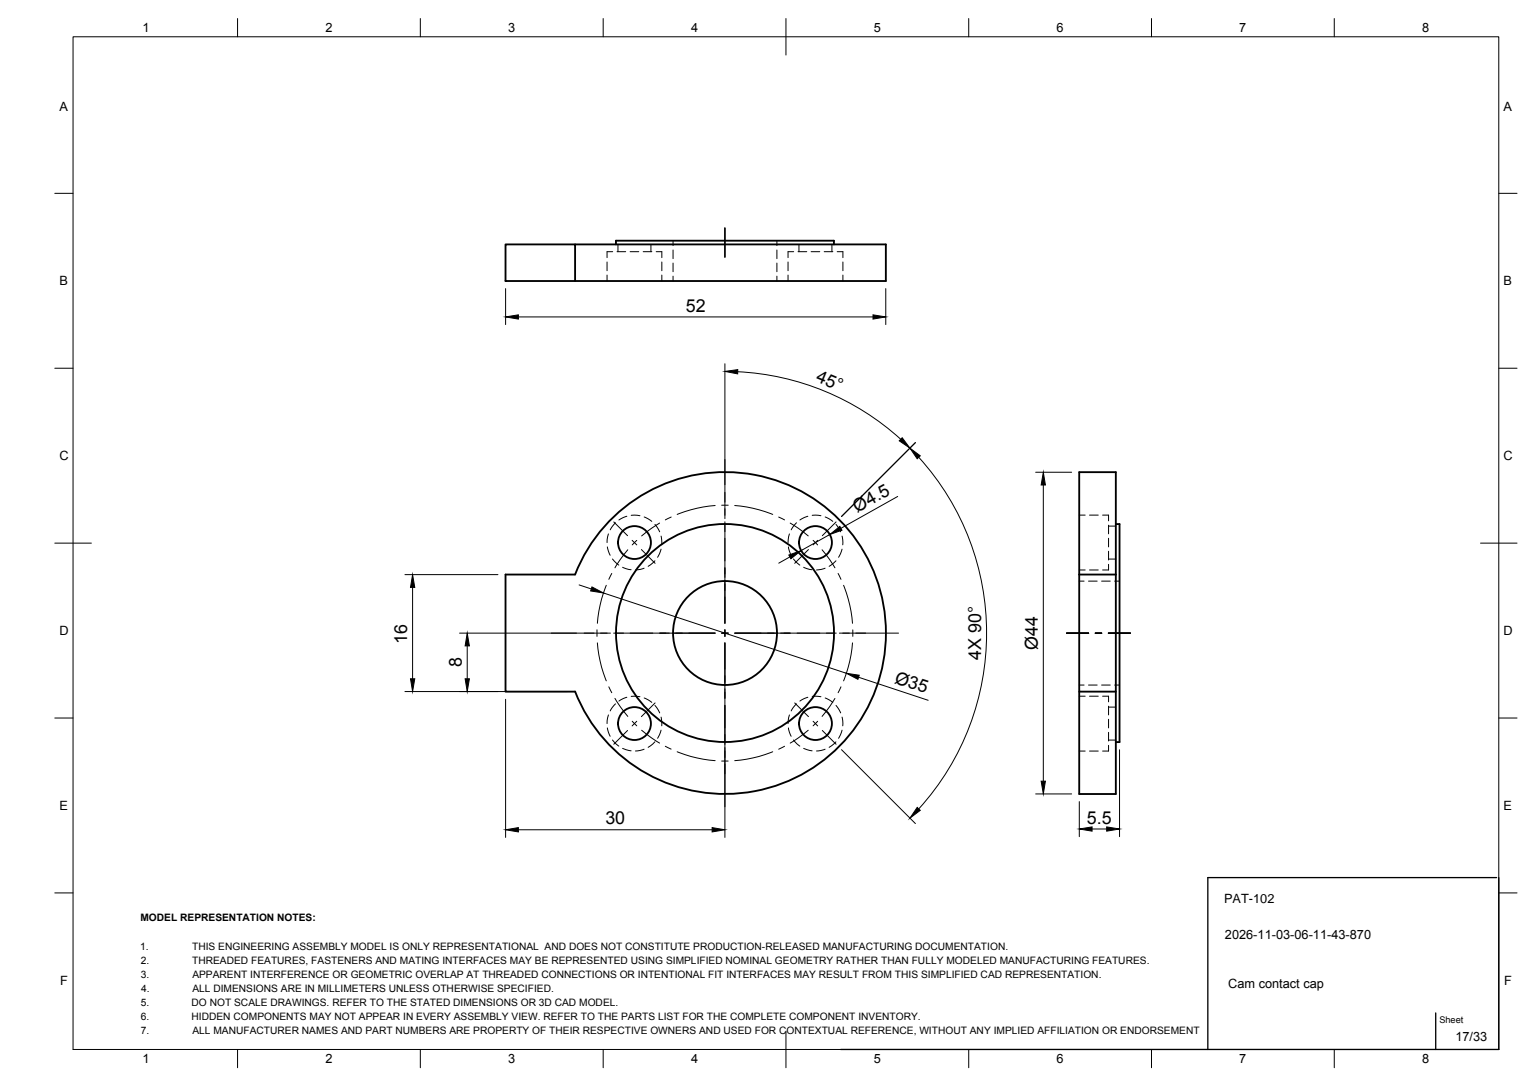
ISO-10303-21;
HEADER;
/* Generated by software containing ST-Developer
 * from STEP Tools, Inc. (www.steptools.com) 
 */

FILE_DESCRIPTION(
/* description */ ('Swing-away clamp arm'),
/* implementation_level */ '2;1');

FILE_NAME(
/* name */ 'Cam contact cap.step',
/* time_stamp */ '2026-10-28T03:26:03-07:00',
/* author */ (''),
/* organization */ (''),
/* preprocessor_version */ 'ST-DEVELOPER v20.2',
/* originating_system */ 'Autodesk Translation Framework v15.17.0.0',
/* authorisation */ '');

FILE_SCHEMA (('AUTOMOTIVE_DESIGN { 1 0 10303 214 3 1 1 }'));
ENDSEC;

DATA;
#10=MECHANICAL_DESIGN_GEOMETRIC_PRESENTATION_REPRESENTATION('',(#304),#10627);
#252=SHAPE_REPRESENTATION_RELATIONSHIP('SRR','None',#10751,#278);
#278=ADVANCED_BREP_SHAPE_REPRESENTATION('',(#337),#10610);
#304=STYLED_ITEM('',(#10951),#337);
#337=MANIFOLD_SOLID_BREP('Body1',#4911);
#416=FACE_BOUND('',#1161,.T.);
#417=FACE_BOUND('',#1164,.T.);
#418=FACE_BOUND('',#1167,.T.);
#419=FACE_BOUND('',#1170,.T.);
#420=FACE_BOUND('',#1180,.T.);
#421=FACE_BOUND('',#1184,.T.);
#422=FACE_BOUND('',#1185,.T.);
#423=FACE_BOUND('',#1186,.T.);
#424=FACE_BOUND('',#1187,.T.);
#425=FACE_BOUND('',#1188,.T.);
#426=FACE_BOUND('',#1190,.T.);
#427=FACE_BOUND('',#1191,.T.);
#428=FACE_BOUND('',#1192,.T.);
#429=FACE_BOUND('',#1193,.T.);
#430=FACE_BOUND('',#1194,.T.);
#563=PLANE('',#5523);
#564=PLANE('',#5528);
#565=PLANE('',#5533);
#566=PLANE('',#5538);
#567=PLANE('',#5548);
#568=PLANE('',#5549);
#569=PLANE('',#5550);
#570=PLANE('',#5554);
#571=PLANE('',#5561);
#572=PLANE('',#5562);
#794=FACE_OUTER_BOUND('',#1159,.T.);
#795=FACE_OUTER_BOUND('',#1160,.T.);
#796=FACE_OUTER_BOUND('',#1162,.T.);
#797=FACE_OUTER_BOUND('',#1163,.T.);
#798=FACE_OUTER_BOUND('',#1165,.T.);
#799=FACE_OUTER_BOUND('',#1166,.T.);
#800=FACE_OUTER_BOUND('',#1168,.T.);
#801=FACE_OUTER_BOUND('',#1169,.T.);
#802=FACE_OUTER_BOUND('',#1171,.T.);
#803=FACE_OUTER_BOUND('',#1172,.T.);
#804=FACE_OUTER_BOUND('',#1173,.T.);
#805=FACE_OUTER_BOUND('',#1174,.T.);
#806=FACE_OUTER_BOUND('',#1175,.T.);
#807=FACE_OUTER_BOUND('',#1176,.T.);
#808=FACE_OUTER_BOUND('',#1177,.T.);
#809=FACE_OUTER_BOUND('',#1178,.T.);
#810=FACE_OUTER_BOUND('',#1179,.T.);
#811=FACE_OUTER_BOUND('',#1181,.T.);
#812=FACE_OUTER_BOUND('',#1182,.T.);
#813=FACE_OUTER_BOUND('',#1183,.T.);
#814=FACE_OUTER_BOUND('',#1189,.T.);
#1159=EDGE_LOOP('',(#3939,#3940,#3941,#3942));
#1160=EDGE_LOOP('',(#3943));
#1161=EDGE_LOOP('',(#3944));
#1162=EDGE_LOOP('',(#3945,#3946,#3947,#3948));
#1163=EDGE_LOOP('',(#3949));
#1164=EDGE_LOOP('',(#3950));
#1165=EDGE_LOOP('',(#3951,#3952,#3953,#3954));
#1166=EDGE_LOOP('',(#3955));
#1167=EDGE_LOOP('',(#3956));
#1168=EDGE_LOOP('',(#3957,#3958,#3959,#3960));
#1169=EDGE_LOOP('',(#3961));
#1170=EDGE_LOOP('',(#3962));
#1171=EDGE_LOOP('',(#3963,#3964,#3965,#3966));
#1172=EDGE_LOOP('',(#3967,#3968,#3969,#3970));
#1173=EDGE_LOOP('',(#3971,#3972,#3973,#3974));
#1174=EDGE_LOOP('',(#3975,#3976,#3977,#3978));
#1175=EDGE_LOOP('',(#3979,#3980,#3981,#3982));
#1176=EDGE_LOOP('',(#3983,#3984,#3985,#3986));
#1177=EDGE_LOOP('',(#3987,#3988,#3989,#3990));
#1178=EDGE_LOOP('',(#3991,#3992,#3993,#3994));
#1179=EDGE_LOOP('',(#3995));
#1180=EDGE_LOOP('',(#3996));
#1181=EDGE_LOOP('',(#3997,#3998,#3999,#4000));
#1182=EDGE_LOOP('',(#4001,#4002,#4003,#4004));
#1183=EDGE_LOOP('',(#4005,#4006,#4007,#4008));
#1184=EDGE_LOOP('',(#4009));
#1185=EDGE_LOOP('',(#4010));
#1186=EDGE_LOOP('',(#4011));
#1187=EDGE_LOOP('',(#4012));
#1188=EDGE_LOOP('',(#4013));
#1189=EDGE_LOOP('',(#4014,#4015,#4016,#4017));
#1190=EDGE_LOOP('',(#4018));
#1191=EDGE_LOOP('',(#4019));
#1192=EDGE_LOOP('',(#4020));
#1193=EDGE_LOOP('',(#4021));
#1194=EDGE_LOOP('',(#4022));
#1563=LINE('',#9559,#1885);
#1564=LINE('',#9568,#1886);
#1565=LINE('',#9577,#1887);
#1566=LINE('',#9586,#1888);
#1567=LINE('',#9594,#1889);
#1568=LINE('',#9598,#1890);
#1569=LINE('',#9602,#1891);
#1570=LINE('',#9606,#1892);
#1571=LINE('',#9610,#1893);
#1572=LINE('',#9612,#1894);
#1573=LINE('',#9614,#1895);
#1574=LINE('',#9615,#1896);
#1575=LINE('',#9619,#1897);
#1576=LINE('',#9621,#1898);
#1577=LINE('',#9623,#1899);
#1578=LINE('',#9624,#1900);
#1579=LINE('',#9626,#1901);
#1580=LINE('',#9627,#1902);
#1581=LINE('',#9632,#1903);
#1582=LINE('',#9640,#1904);
#1885=VECTOR('',#6680,0.375);
#1886=VECTOR('',#6691,0.375);
#1887=VECTOR('',#6702,0.375);
#1888=VECTOR('',#6713,0.375);
#1889=VECTOR('',#6724,0.225);
#1890=VECTOR('',#6729,0.225);
#1891=VECTOR('',#6734,0.225);
#1892=VECTOR('',#6739,0.225);
#1893=VECTOR('',#6742,1.);
#1894=VECTOR('',#6743,1.);
#1895=VECTOR('',#6744,1.);
#1896=VECTOR('',#6745,1.);
#1897=VECTOR('',#6748,1.);
#1898=VECTOR('',#6749,1.);
#1899=VECTOR('',#6750,1.);
#1900=VECTOR('',#6751,1.);
#1901=VECTOR('',#6754,1.);
#1902=VECTOR('',#6755,1.);
#1903=VECTOR('',#6760,1.49);
#1904=VECTOR('',#6771,0.71);
#2111=CIRCLE('',#5521,0.375);
#2112=CIRCLE('',#5522,0.375);
#2113=CIRCLE('',#5524,0.225);
#2114=CIRCLE('',#5526,0.375);
#2115=CIRCLE('',#5527,0.375);
#2116=CIRCLE('',#5529,0.225);
#2117=CIRCLE('',#5531,0.375);
#2118=CIRCLE('',#5532,0.375);
#2119=CIRCLE('',#5534,0.225);
#2120=CIRCLE('',#5536,0.375);
#2121=CIRCLE('',#5537,0.375);
#2122=CIRCLE('',#5539,0.225);
#2123=CIRCLE('',#5541,0.225);
#2124=CIRCLE('',#5543,0.225);
#2125=CIRCLE('',#5545,0.225);
#2126=CIRCLE('',#5547,0.225);
#2127=CIRCLE('',#5552,1.49);
#2128=CIRCLE('',#5553,1.49);
#2129=CIRCLE('',#5555,0.71);
#2130=CIRCLE('',#5557,0.71);
#2131=CIRCLE('',#5559,2.2);
#2132=CIRCLE('',#5560,2.2);
#2480=VERTEX_POINT('',#9556);
#2481=VERTEX_POINT('',#9558);
#2482=VERTEX_POINT('',#9562);
#2483=VERTEX_POINT('',#9565);
#2484=VERTEX_POINT('',#9567);
#2485=VERTEX_POINT('',#9571);
#2486=VERTEX_POINT('',#9574);
#2487=VERTEX_POINT('',#9576);
#2488=VERTEX_POINT('',#9580);
#2489=VERTEX_POINT('',#9583);
#2490=VERTEX_POINT('',#9585);
#2491=VERTEX_POINT('',#9589);
#2492=VERTEX_POINT('',#9592);
#2493=VERTEX_POINT('',#9596);
#2494=VERTEX_POINT('',#9600);
#2495=VERTEX_POINT('',#9604);
#2496=VERTEX_POINT('',#9608);
#2497=VERTEX_POINT('',#9609);
#2498=VERTEX_POINT('',#9611);
#2499=VERTEX_POINT('',#9613);
#2500=VERTEX_POINT('',#9617);
#2501=VERTEX_POINT('',#9618);
#2502=VERTEX_POINT('',#9620);
#2503=VERTEX_POINT('',#9622);
#2504=VERTEX_POINT('',#9629);
#2505=VERTEX_POINT('',#9631);
#2506=VERTEX_POINT('',#9635);
#2507=VERTEX_POINT('',#9638);
#3002=EDGE_CURVE('',#2480,#2480,#2111,.T.);
#3003=EDGE_CURVE('',#2480,#2481,#1563,.T.);
#3004=EDGE_CURVE('',#2481,#2481,#2112,.T.);
#3005=EDGE_CURVE('',#2482,#2482,#2113,.T.);
#3006=EDGE_CURVE('',#2483,#2483,#2114,.T.);
#3007=EDGE_CURVE('',#2483,#2484,#1564,.T.);
#3008=EDGE_CURVE('',#2484,#2484,#2115,.T.);
#3009=EDGE_CURVE('',#2485,#2485,#2116,.T.);
#3010=EDGE_CURVE('',#2486,#2486,#2117,.T.);
#3011=EDGE_CURVE('',#2486,#2487,#1565,.T.);
#3012=EDGE_CURVE('',#2487,#2487,#2118,.T.);
#3013=EDGE_CURVE('',#2488,#2488,#2119,.T.);
#3014=EDGE_CURVE('',#2489,#2489,#2120,.T.);
#3015=EDGE_CURVE('',#2489,#2490,#1566,.T.);
#3016=EDGE_CURVE('',#2490,#2490,#2121,.T.);
#3017=EDGE_CURVE('',#2491,#2491,#2122,.T.);
#3018=EDGE_CURVE('',#2492,#2492,#2123,.T.);
#3019=EDGE_CURVE('',#2492,#2482,#1567,.T.);
#3020=EDGE_CURVE('',#2493,#2493,#2124,.T.);
#3021=EDGE_CURVE('',#2493,#2485,#1568,.T.);
#3022=EDGE_CURVE('',#2494,#2494,#2125,.T.);
#3023=EDGE_CURVE('',#2494,#2488,#1569,.T.);
#3024=EDGE_CURVE('',#2495,#2495,#2126,.T.);
#3025=EDGE_CURVE('',#2495,#2491,#1570,.T.);
#3026=EDGE_CURVE('',#2496,#2497,#1571,.T.);
#3027=EDGE_CURVE('',#2498,#2496,#1572,.T.);
#3028=EDGE_CURVE('',#2499,#2498,#1573,.T.);
#3029=EDGE_CURVE('',#2499,#2497,#1574,.T.);
#3030=EDGE_CURVE('',#2500,#2501,#1575,.T.);
#3031=EDGE_CURVE('',#2500,#2502,#1576,.T.);
#3032=EDGE_CURVE('',#2502,#2503,#1577,.T.);
#3033=EDGE_CURVE('',#2501,#2503,#1578,.T.);
#3034=EDGE_CURVE('',#2502,#2499,#1579,.T.);
#3035=EDGE_CURVE('',#2503,#2498,#1580,.T.);
#3036=EDGE_CURVE('',#2504,#2504,#2127,.T.);
#3037=EDGE_CURVE('',#2504,#2505,#1581,.T.);
#3038=EDGE_CURVE('',#2505,#2505,#2128,.T.);
#3039=EDGE_CURVE('',#2506,#2506,#2129,.T.);
#3040=EDGE_CURVE('',#2507,#2507,#2130,.T.);
#3041=EDGE_CURVE('',#2507,#2506,#1582,.T.);
#3042=EDGE_CURVE('',#2497,#2500,#2131,.T.);
#3043=EDGE_CURVE('',#2496,#2501,#2132,.T.);
#3939=ORIENTED_EDGE('',*,*,#3002,.F.);
#3940=ORIENTED_EDGE('',*,*,#3003,.T.);
#3941=ORIENTED_EDGE('',*,*,#3004,.F.);
#3942=ORIENTED_EDGE('',*,*,#3003,.F.);
#3943=ORIENTED_EDGE('',*,*,#3002,.T.);
#3944=ORIENTED_EDGE('',*,*,#3005,.F.);
#3945=ORIENTED_EDGE('',*,*,#3006,.F.);
#3946=ORIENTED_EDGE('',*,*,#3007,.T.);
#3947=ORIENTED_EDGE('',*,*,#3008,.F.);
#3948=ORIENTED_EDGE('',*,*,#3007,.F.);
#3949=ORIENTED_EDGE('',*,*,#3006,.T.);
#3950=ORIENTED_EDGE('',*,*,#3009,.F.);
#3951=ORIENTED_EDGE('',*,*,#3010,.F.);
#3952=ORIENTED_EDGE('',*,*,#3011,.T.);
#3953=ORIENTED_EDGE('',*,*,#3012,.F.);
#3954=ORIENTED_EDGE('',*,*,#3011,.F.);
#3955=ORIENTED_EDGE('',*,*,#3010,.T.);
#3956=ORIENTED_EDGE('',*,*,#3013,.F.);
#3957=ORIENTED_EDGE('',*,*,#3014,.F.);
#3958=ORIENTED_EDGE('',*,*,#3015,.T.);
#3959=ORIENTED_EDGE('',*,*,#3016,.F.);
#3960=ORIENTED_EDGE('',*,*,#3015,.F.);
#3961=ORIENTED_EDGE('',*,*,#3014,.T.);
#3962=ORIENTED_EDGE('',*,*,#3017,.F.);
#3963=ORIENTED_EDGE('',*,*,#3018,.F.);
#3964=ORIENTED_EDGE('',*,*,#3019,.T.);
#3965=ORIENTED_EDGE('',*,*,#3005,.T.);
#3966=ORIENTED_EDGE('',*,*,#3019,.F.);
#3967=ORIENTED_EDGE('',*,*,#3020,.F.);
#3968=ORIENTED_EDGE('',*,*,#3021,.T.);
#3969=ORIENTED_EDGE('',*,*,#3009,.T.);
#3970=ORIENTED_EDGE('',*,*,#3021,.F.);
#3971=ORIENTED_EDGE('',*,*,#3022,.F.);
#3972=ORIENTED_EDGE('',*,*,#3023,.T.);
#3973=ORIENTED_EDGE('',*,*,#3013,.T.);
#3974=ORIENTED_EDGE('',*,*,#3023,.F.);
#3975=ORIENTED_EDGE('',*,*,#3024,.F.);
#3976=ORIENTED_EDGE('',*,*,#3025,.T.);
#3977=ORIENTED_EDGE('',*,*,#3017,.T.);
#3978=ORIENTED_EDGE('',*,*,#3025,.F.);
#3979=ORIENTED_EDGE('',*,*,#3026,.F.);
#3980=ORIENTED_EDGE('',*,*,#3027,.F.);
#3981=ORIENTED_EDGE('',*,*,#3028,.F.);
#3982=ORIENTED_EDGE('',*,*,#3029,.T.);
#3983=ORIENTED_EDGE('',*,*,#3030,.F.);
#3984=ORIENTED_EDGE('',*,*,#3031,.T.);
#3985=ORIENTED_EDGE('',*,*,#3032,.T.);
#3986=ORIENTED_EDGE('',*,*,#3033,.F.);
#3987=ORIENTED_EDGE('',*,*,#3034,.T.);
#3988=ORIENTED_EDGE('',*,*,#3028,.T.);
#3989=ORIENTED_EDGE('',*,*,#3035,.F.);
#3990=ORIENTED_EDGE('',*,*,#3032,.F.);
#3991=ORIENTED_EDGE('',*,*,#3036,.F.);
#3992=ORIENTED_EDGE('',*,*,#3037,.T.);
#3993=ORIENTED_EDGE('',*,*,#3038,.T.);
#3994=ORIENTED_EDGE('',*,*,#3037,.F.);
#3995=ORIENTED_EDGE('',*,*,#3038,.F.);
#3996=ORIENTED_EDGE('',*,*,#3039,.F.);
#3997=ORIENTED_EDGE('',*,*,#3040,.F.);
#3998=ORIENTED_EDGE('',*,*,#3041,.T.);
#3999=ORIENTED_EDGE('',*,*,#3039,.T.);
#4000=ORIENTED_EDGE('',*,*,#3041,.F.);
#4001=ORIENTED_EDGE('',*,*,#3026,.T.);
#4002=ORIENTED_EDGE('',*,*,#3042,.T.);
#4003=ORIENTED_EDGE('',*,*,#3030,.T.);
#4004=ORIENTED_EDGE('',*,*,#3043,.F.);
#4005=ORIENTED_EDGE('',*,*,#3043,.T.);
#4006=ORIENTED_EDGE('',*,*,#3033,.T.);
#4007=ORIENTED_EDGE('',*,*,#3035,.T.);
#4008=ORIENTED_EDGE('',*,*,#3027,.T.);
#4009=ORIENTED_EDGE('',*,*,#3040,.T.);
#4010=ORIENTED_EDGE('',*,*,#3016,.T.);
#4011=ORIENTED_EDGE('',*,*,#3012,.T.);
#4012=ORIENTED_EDGE('',*,*,#3008,.T.);
#4013=ORIENTED_EDGE('',*,*,#3004,.T.);
#4014=ORIENTED_EDGE('',*,*,#3042,.F.);
#4015=ORIENTED_EDGE('',*,*,#3029,.F.);
#4016=ORIENTED_EDGE('',*,*,#3034,.F.);
#4017=ORIENTED_EDGE('',*,*,#3031,.F.);
#4018=ORIENTED_EDGE('',*,*,#3036,.T.);
#4019=ORIENTED_EDGE('',*,*,#3024,.T.);
#4020=ORIENTED_EDGE('',*,*,#3022,.T.);
#4021=ORIENTED_EDGE('',*,*,#3020,.T.);
#4022=ORIENTED_EDGE('',*,*,#3018,.T.);
#4545=CYLINDRICAL_SURFACE('',#5520,0.375);
#4546=CYLINDRICAL_SURFACE('',#5525,0.375);
#4547=CYLINDRICAL_SURFACE('',#5530,0.375);
#4548=CYLINDRICAL_SURFACE('',#5535,0.375);
#4549=CYLINDRICAL_SURFACE('',#5540,0.225);
#4550=CYLINDRICAL_SURFACE('',#5542,0.225);
#4551=CYLINDRICAL_SURFACE('',#5544,0.225);
#4552=CYLINDRICAL_SURFACE('',#5546,0.225);
#4553=CYLINDRICAL_SURFACE('',#5551,1.49);
#4554=CYLINDRICAL_SURFACE('',#5556,0.71);
#4555=CYLINDRICAL_SURFACE('',#5558,2.2);
#4749=ADVANCED_FACE('',(#794),#4545,.F.);
#4750=ADVANCED_FACE('',(#795,#416),#563,.T.);
#4751=ADVANCED_FACE('',(#796),#4546,.F.);
#4752=ADVANCED_FACE('',(#797,#417),#564,.T.);
#4753=ADVANCED_FACE('',(#798),#4547,.F.);
#4754=ADVANCED_FACE('',(#799,#418),#565,.T.);
#4755=ADVANCED_FACE('',(#800),#4548,.F.);
#4756=ADVANCED_FACE('',(#801,#419),#566,.T.);
#4757=ADVANCED_FACE('',(#802),#4549,.F.);
#4758=ADVANCED_FACE('',(#803),#4550,.F.);
#4759=ADVANCED_FACE('',(#804),#4551,.F.);
#4760=ADVANCED_FACE('',(#805),#4552,.F.);
#4761=ADVANCED_FACE('',(#806),#567,.T.);
#4762=ADVANCED_FACE('',(#807),#568,.T.);
#4763=ADVANCED_FACE('',(#808),#569,.T.);
#4764=ADVANCED_FACE('',(#809),#4553,.T.);
#4765=ADVANCED_FACE('',(#810,#420),#570,.F.);
#4766=ADVANCED_FACE('',(#811),#4554,.F.);
#4767=ADVANCED_FACE('',(#812),#4555,.T.);
#4768=ADVANCED_FACE('',(#813,#421,#422,#423,#424,#425),#571,.T.);
#4769=ADVANCED_FACE('',(#814,#426,#427,#428,#429,#430),#572,.F.);
#4911=CLOSED_SHELL('',(#4749,#4750,#4751,#4752,#4753,#4754,#4755,#4756,
#4757,#4758,#4759,#4760,#4761,#4762,#4763,#4764,#4765,#4766,#4767,#4768,
#4769));
#5519=AXIS2_PLACEMENT_3D('',#9554,#6674,#6675);
#5520=AXIS2_PLACEMENT_3D('',#9555,#6676,#6677);
#5521=AXIS2_PLACEMENT_3D('',#9557,#6678,#6679);
#5522=AXIS2_PLACEMENT_3D('',#9560,#6681,#6682);
#5523=AXIS2_PLACEMENT_3D('',#9561,#6683,#6684);
#5524=AXIS2_PLACEMENT_3D('',#9563,#6685,#6686);
#5525=AXIS2_PLACEMENT_3D('',#9564,#6687,#6688);
#5526=AXIS2_PLACEMENT_3D('',#9566,#6689,#6690);
#5527=AXIS2_PLACEMENT_3D('',#9569,#6692,#6693);
#5528=AXIS2_PLACEMENT_3D('',#9570,#6694,#6695);
#5529=AXIS2_PLACEMENT_3D('',#9572,#6696,#6697);
#5530=AXIS2_PLACEMENT_3D('',#9573,#6698,#6699);
#5531=AXIS2_PLACEMENT_3D('',#9575,#6700,#6701);
#5532=AXIS2_PLACEMENT_3D('',#9578,#6703,#6704);
#5533=AXIS2_PLACEMENT_3D('',#9579,#6705,#6706);
#5534=AXIS2_PLACEMENT_3D('',#9581,#6707,#6708);
#5535=AXIS2_PLACEMENT_3D('',#9582,#6709,#6710);
#5536=AXIS2_PLACEMENT_3D('',#9584,#6711,#6712);
#5537=AXIS2_PLACEMENT_3D('',#9587,#6714,#6715);
#5538=AXIS2_PLACEMENT_3D('',#9588,#6716,#6717);
#5539=AXIS2_PLACEMENT_3D('',#9590,#6718,#6719);
#5540=AXIS2_PLACEMENT_3D('',#9591,#6720,#6721);
#5541=AXIS2_PLACEMENT_3D('',#9593,#6722,#6723);
#5542=AXIS2_PLACEMENT_3D('',#9595,#6725,#6726);
#5543=AXIS2_PLACEMENT_3D('',#9597,#6727,#6728);
#5544=AXIS2_PLACEMENT_3D('',#9599,#6730,#6731);
#5545=AXIS2_PLACEMENT_3D('',#9601,#6732,#6733);
#5546=AXIS2_PLACEMENT_3D('',#9603,#6735,#6736);
#5547=AXIS2_PLACEMENT_3D('',#9605,#6737,#6738);
#5548=AXIS2_PLACEMENT_3D('',#9607,#6740,#6741);
#5549=AXIS2_PLACEMENT_3D('',#9616,#6746,#6747);
#5550=AXIS2_PLACEMENT_3D('',#9625,#6752,#6753);
#5551=AXIS2_PLACEMENT_3D('',#9628,#6756,#6757);
#5552=AXIS2_PLACEMENT_3D('',#9630,#6758,#6759);
#5553=AXIS2_PLACEMENT_3D('',#9633,#6761,#6762);
#5554=AXIS2_PLACEMENT_3D('',#9634,#6763,#6764);
#5555=AXIS2_PLACEMENT_3D('',#9636,#6765,#6766);
#5556=AXIS2_PLACEMENT_3D('',#9637,#6767,#6768);
#5557=AXIS2_PLACEMENT_3D('',#9639,#6769,#6770);
#5558=AXIS2_PLACEMENT_3D('',#9641,#6772,#6773);
#5559=AXIS2_PLACEMENT_3D('',#9642,#6774,#6775);
#5560=AXIS2_PLACEMENT_3D('',#9643,#6776,#6777);
#5561=AXIS2_PLACEMENT_3D('',#9644,#6778,#6779);
#5562=AXIS2_PLACEMENT_3D('',#9645,#6780,#6781);
#6674=DIRECTION('axis',(0.,0.,1.));
#6675=DIRECTION('refdir',(1.,0.,0.));
#6676=DIRECTION('center_axis',(0.,0.,1.));
#6677=DIRECTION('ref_axis',(1.,0.,0.));
#6678=DIRECTION('center_axis',(0.,0.,1.));
#6679=DIRECTION('ref_axis',(1.,0.,0.));
#6680=DIRECTION('',(0.,0.,1.));
#6681=DIRECTION('center_axis',(0.,0.,-1.));
#6682=DIRECTION('ref_axis',(1.,0.,0.));
#6683=DIRECTION('center_axis',(0.,0.,1.));
#6684=DIRECTION('ref_axis',(1.,0.,0.));
#6685=DIRECTION('center_axis',(0.,0.,1.));
#6686=DIRECTION('ref_axis',(1.,0.,0.));
#6687=DIRECTION('center_axis',(0.,0.,1.));
#6688=DIRECTION('ref_axis',(1.,0.,0.));
#6689=DIRECTION('center_axis',(0.,0.,1.));
#6690=DIRECTION('ref_axis',(1.,0.,0.));
#6691=DIRECTION('',(0.,0.,1.));
#6692=DIRECTION('center_axis',(0.,0.,-1.));
#6693=DIRECTION('ref_axis',(1.,0.,0.));
#6694=DIRECTION('center_axis',(0.,0.,1.));
#6695=DIRECTION('ref_axis',(1.,0.,0.));
#6696=DIRECTION('center_axis',(0.,0.,1.));
#6697=DIRECTION('ref_axis',(1.,0.,0.));
#6698=DIRECTION('center_axis',(0.,0.,1.));
#6699=DIRECTION('ref_axis',(1.,0.,0.));
#6700=DIRECTION('center_axis',(0.,0.,1.));
#6701=DIRECTION('ref_axis',(1.,0.,0.));
#6702=DIRECTION('',(0.,0.,1.));
#6703=DIRECTION('center_axis',(0.,0.,-1.));
#6704=DIRECTION('ref_axis',(1.,0.,0.));
#6705=DIRECTION('center_axis',(0.,0.,1.));
#6706=DIRECTION('ref_axis',(1.,0.,0.));
#6707=DIRECTION('center_axis',(0.,0.,1.));
#6708=DIRECTION('ref_axis',(1.,0.,0.));
#6709=DIRECTION('center_axis',(0.,0.,1.));
#6710=DIRECTION('ref_axis',(1.,0.,0.));
#6711=DIRECTION('center_axis',(0.,0.,1.));
#6712=DIRECTION('ref_axis',(1.,0.,0.));
#6713=DIRECTION('',(0.,0.,1.));
#6714=DIRECTION('center_axis',(0.,0.,-1.));
#6715=DIRECTION('ref_axis',(1.,0.,0.));
#6716=DIRECTION('center_axis',(0.,0.,1.));
#6717=DIRECTION('ref_axis',(1.,0.,0.));
#6718=DIRECTION('center_axis',(0.,0.,1.));
#6719=DIRECTION('ref_axis',(1.,0.,0.));
#6720=DIRECTION('center_axis',(0.,0.,1.));
#6721=DIRECTION('ref_axis',(1.,0.,0.));
#6722=DIRECTION('center_axis',(0.,0.,1.));
#6723=DIRECTION('ref_axis',(1.,0.,0.));
#6724=DIRECTION('',(0.,0.,1.));
#6725=DIRECTION('center_axis',(0.,0.,1.));
#6726=DIRECTION('ref_axis',(1.,0.,0.));
#6727=DIRECTION('center_axis',(0.,0.,1.));
#6728=DIRECTION('ref_axis',(1.,0.,0.));
#6729=DIRECTION('',(0.,0.,1.));
#6730=DIRECTION('center_axis',(0.,0.,1.));
#6731=DIRECTION('ref_axis',(1.,0.,0.));
#6732=DIRECTION('center_axis',(0.,0.,1.));
#6733=DIRECTION('ref_axis',(1.,0.,0.));
#6734=DIRECTION('',(0.,0.,1.));
#6735=DIRECTION('center_axis',(0.,0.,1.));
#6736=DIRECTION('ref_axis',(1.,0.,0.));
#6737=DIRECTION('center_axis',(0.,0.,1.));
#6738=DIRECTION('ref_axis',(1.,0.,0.));
#6739=DIRECTION('',(0.,0.,1.));
#6740=DIRECTION('center_axis',(0.,1.,0.));
#6741=DIRECTION('ref_axis',(-1.,0.,0.));
#6742=DIRECTION('',(0.,0.,-1.));
#6743=DIRECTION('',(-1.,0.,0.));
#6744=DIRECTION('',(0.,0.,1.));
#6745=DIRECTION('',(-1.,0.,0.));
#6746=DIRECTION('center_axis',(0.,-1.,0.));
#6747=DIRECTION('ref_axis',(1.,0.,0.));
#6748=DIRECTION('',(0.,0.,1.));
#6749=DIRECTION('',(1.,0.,0.));
#6750=DIRECTION('',(0.,0.,1.));
#6751=DIRECTION('',(1.,0.,0.));
#6752=DIRECTION('center_axis',(1.,0.,0.));
#6753=DIRECTION('ref_axis',(0.,1.,0.));
#6754=DIRECTION('',(0.,1.,0.));
#6755=DIRECTION('',(0.,1.,0.));
#6756=DIRECTION('center_axis',(0.,0.,1.));
#6757=DIRECTION('ref_axis',(1.,0.,0.));
#6758=DIRECTION('center_axis',(0.,0.,1.));
#6759=DIRECTION('ref_axis',(1.,0.,0.));
#6760=DIRECTION('',(0.,0.,-1.));
#6761=DIRECTION('center_axis',(0.,0.,1.));
#6762=DIRECTION('ref_axis',(1.,0.,0.));
#6763=DIRECTION('center_axis',(0.,0.,1.));
#6764=DIRECTION('ref_axis',(1.,0.,0.));
#6765=DIRECTION('center_axis',(0.,0.,-1.));
#6766=DIRECTION('ref_axis',(1.,0.,0.));
#6767=DIRECTION('center_axis',(0.,0.,1.));
#6768=DIRECTION('ref_axis',(1.,0.,0.));
#6769=DIRECTION('center_axis',(0.,0.,-1.));
#6770=DIRECTION('ref_axis',(1.,0.,0.));
#6771=DIRECTION('',(0.,0.,-1.));
#6772=DIRECTION('center_axis',(0.,0.,1.));
#6773=DIRECTION('ref_axis',(-1.,1.22464679914735E-16,0.));
#6774=DIRECTION('center_axis',(0.,0.,1.));
#6775=DIRECTION('ref_axis',(1.,0.,0.));
#6776=DIRECTION('center_axis',(0.,0.,1.));
#6777=DIRECTION('ref_axis',(1.,0.,0.));
#6778=DIRECTION('center_axis',(0.,0.,1.));
#6779=DIRECTION('ref_axis',(1.,0.,0.));
#6780=DIRECTION('center_axis',(0.,0.,1.));
#6781=DIRECTION('ref_axis',(1.,0.,0.));
#9554=CARTESIAN_POINT('',(0.,0.,0.));
#9555=CARTESIAN_POINT('Origin',(-1.23743686707646,-1.23743686707646,9.1));
#9556=CARTESIAN_POINT('',(-1.61243686707646,-1.23743686707646,9.1));
#9557=CARTESIAN_POINT('Origin',(-1.23743686707646,-1.23743686707646,9.1));
#9558=CARTESIAN_POINT('',(-1.61243686707646,-1.23743686707646,9.5));
#9559=CARTESIAN_POINT('',(-1.61243686707646,-1.23743686707646,9.1));
#9560=CARTESIAN_POINT('Origin',(-1.23743686707646,-1.23743686707646,9.5));
#9561=CARTESIAN_POINT('Origin',(-1.23743686707646,-1.23743686707646,9.1));
#9562=CARTESIAN_POINT('',(-1.46243686707646,-1.23743686707646,9.1));
#9563=CARTESIAN_POINT('Origin',(-1.23743686707646,-1.23743686707646,9.1));
#9564=CARTESIAN_POINT('Origin',(-1.23743686707646,1.23743686707646,9.1));
#9565=CARTESIAN_POINT('',(-1.61243686707646,1.23743686707646,9.1));
#9566=CARTESIAN_POINT('Origin',(-1.23743686707646,1.23743686707646,9.1));
#9567=CARTESIAN_POINT('',(-1.61243686707646,1.23743686707646,9.5));
#9568=CARTESIAN_POINT('',(-1.61243686707646,1.23743686707646,9.1));
#9569=CARTESIAN_POINT('Origin',(-1.23743686707646,1.23743686707646,9.5));
#9570=CARTESIAN_POINT('Origin',(-1.23743686707646,1.23743686707646,9.1));
#9571=CARTESIAN_POINT('',(-1.46243686707646,1.23743686707646,9.1));
#9572=CARTESIAN_POINT('Origin',(-1.23743686707646,1.23743686707646,9.1));
#9573=CARTESIAN_POINT('Origin',(1.23743686707646,1.23743686707646,9.1));
#9574=CARTESIAN_POINT('',(0.862436867076458,1.23743686707646,9.1));
#9575=CARTESIAN_POINT('Origin',(1.23743686707646,1.23743686707646,9.1));
#9576=CARTESIAN_POINT('',(0.862436867076458,1.23743686707646,9.5));
#9577=CARTESIAN_POINT('',(0.862436867076458,1.23743686707646,9.1));
#9578=CARTESIAN_POINT('Origin',(1.23743686707646,1.23743686707646,9.5));
#9579=CARTESIAN_POINT('Origin',(1.23743686707646,1.23743686707646,9.1));
#9580=CARTESIAN_POINT('',(1.01243686707646,1.23743686707646,9.1));
#9581=CARTESIAN_POINT('Origin',(1.23743686707646,1.23743686707646,9.1));
#9582=CARTESIAN_POINT('Origin',(1.23743686707646,-1.23743686707646,9.1));
#9583=CARTESIAN_POINT('',(0.862436867076458,-1.23743686707646,9.1));
#9584=CARTESIAN_POINT('Origin',(1.23743686707646,-1.23743686707646,9.1));
#9585=CARTESIAN_POINT('',(0.862436867076458,-1.23743686707646,9.5));
#9586=CARTESIAN_POINT('',(0.862436867076458,-1.23743686707646,9.1));
#9587=CARTESIAN_POINT('Origin',(1.23743686707646,-1.23743686707646,9.5));
#9588=CARTESIAN_POINT('Origin',(1.23743686707646,-1.23743686707646,9.1));
#9589=CARTESIAN_POINT('',(1.01243686707646,-1.23743686707646,9.1));
#9590=CARTESIAN_POINT('Origin',(1.23743686707646,-1.23743686707646,9.1));
#9591=CARTESIAN_POINT('Origin',(-1.23743686707646,-1.23743686707646,8.9));
#9592=CARTESIAN_POINT('',(-1.46243686707646,-1.23743686707646,9.));
#9593=CARTESIAN_POINT('Origin',(-1.23743686707646,-1.23743686707646,9.));
#9594=CARTESIAN_POINT('',(-1.46243686707646,-1.23743686707646,8.9));
#9595=CARTESIAN_POINT('Origin',(-1.23743686707646,1.23743686707646,8.9));
#9596=CARTESIAN_POINT('',(-1.46243686707646,1.23743686707646,9.));
#9597=CARTESIAN_POINT('Origin',(-1.23743686707646,1.23743686707646,9.));
#9598=CARTESIAN_POINT('',(-1.46243686707646,1.23743686707646,8.9));
#9599=CARTESIAN_POINT('Origin',(1.23743686707646,1.23743686707646,8.9));
#9600=CARTESIAN_POINT('',(1.01243686707646,1.23743686707646,9.));
#9601=CARTESIAN_POINT('Origin',(1.23743686707646,1.23743686707646,9.));
#9602=CARTESIAN_POINT('',(1.01243686707646,1.23743686707646,8.9));
#9603=CARTESIAN_POINT('Origin',(1.23743686707646,-1.23743686707646,8.9));
#9604=CARTESIAN_POINT('',(1.01243686707646,-1.23743686707646,9.));
#9605=CARTESIAN_POINT('Origin',(1.23743686707646,-1.23743686707646,9.));
#9606=CARTESIAN_POINT('',(1.01243686707646,-1.23743686707646,8.9));
#9607=CARTESIAN_POINT('Origin',(3.,0.8,9.));
#9608=CARTESIAN_POINT('',(2.04939015319192,0.8,9.5));
#9609=CARTESIAN_POINT('',(2.04939015319192,0.8,9.));
#9610=CARTESIAN_POINT('',(2.04939015319192,0.8,9.));
#9611=CARTESIAN_POINT('',(3.,0.8,9.5));
#9612=CARTESIAN_POINT('',(3.,0.8,9.5));
#9613=CARTESIAN_POINT('',(3.,0.8,9.));
#9614=CARTESIAN_POINT('',(3.,0.8,9.));
#9615=CARTESIAN_POINT('',(3.,0.8,9.));
#9616=CARTESIAN_POINT('Origin',(1.2,-0.8,9.));
#9617=CARTESIAN_POINT('',(2.04939015319192,-0.8,9.));
#9618=CARTESIAN_POINT('',(2.04939015319192,-0.8,9.5));
#9619=CARTESIAN_POINT('',(2.04939015319192,-0.8,9.));
#9620=CARTESIAN_POINT('',(3.,-0.8,9.));
#9621=CARTESIAN_POINT('',(1.2,-0.8,9.));
#9622=CARTESIAN_POINT('',(3.,-0.8,9.5));
#9623=CARTESIAN_POINT('',(3.,-0.8,9.));
#9624=CARTESIAN_POINT('',(1.2,-0.8,9.5));
#9625=CARTESIAN_POINT('Origin',(3.,-0.8,9.));
#9626=CARTESIAN_POINT('',(3.,-0.8,9.));
#9627=CARTESIAN_POINT('',(3.,-0.8,9.5));
#9628=CARTESIAN_POINT('Origin',(0.,0.,8.95));
#9629=CARTESIAN_POINT('',(-1.49,-1.82472373072956E-16,9.));
#9630=CARTESIAN_POINT('Origin',(0.,0.,9.));
#9631=CARTESIAN_POINT('',(-1.49,-1.82472373072956E-16,8.95));
#9632=CARTESIAN_POINT('',(-1.49,-1.82472373072956E-16,8.95));
#9633=CARTESIAN_POINT('Origin',(0.,0.,8.95));
#9634=CARTESIAN_POINT('Origin',(0.,0.,8.95));
#9635=CARTESIAN_POINT('',(-0.71,-8.69499227394621E-17,8.95));
#9636=CARTESIAN_POINT('Origin',(0.,0.,8.95));
#9637=CARTESIAN_POINT('Origin',(0.,0.,9.));
#9638=CARTESIAN_POINT('',(-0.71,-8.69499227394621E-17,9.5));
#9639=CARTESIAN_POINT('Origin',(0.,0.,9.5));
#9640=CARTESIAN_POINT('',(-0.71,-8.69499227394621E-17,9.));
#9641=CARTESIAN_POINT('Origin',(0.,0.,9.));
#9642=CARTESIAN_POINT('Origin',(0.,0.,9.));
#9643=CARTESIAN_POINT('Origin',(0.,0.,9.5));
#9644=CARTESIAN_POINT('Origin',(0.,0.,9.5));
#9645=CARTESIAN_POINT('Origin',(0.,0.,9.));
#10578=UNCERTAINTY_MEASURE_WITH_UNIT(LENGTH_MEASURE(0.001),#10628,
'DISTANCE_ACCURACY_VALUE',
'Maximum model space distance between geometric entities at asserted c
onnectivities');
#10595=UNCERTAINTY_MEASURE_WITH_UNIT(LENGTH_MEASURE(0.001),#10628,
'DISTANCE_ACCURACY_VALUE',
'Maximum model space distance between geometric entities at asserted c
onnectivities');
#10610=(
GEOMETRIC_REPRESENTATION_CONTEXT(3)
GLOBAL_UNCERTAINTY_ASSIGNED_CONTEXT((#10578))
GLOBAL_UNIT_ASSIGNED_CONTEXT((#10628,#10630,#10631))
REPRESENTATION_CONTEXT('','3D')
);
#10627=(
GEOMETRIC_REPRESENTATION_CONTEXT(3)
GLOBAL_UNCERTAINTY_ASSIGNED_CONTEXT((#10595))
GLOBAL_UNIT_ASSIGNED_CONTEXT((#10628,#10630,#10631))
REPRESENTATION_CONTEXT('','3D')
);
#10628=(
LENGTH_UNIT()
NAMED_UNIT(*)
SI_UNIT(.CENTI.,.METRE.)
);
#10630=(
NAMED_UNIT(*)
PLANE_ANGLE_UNIT()
SI_UNIT($,.RADIAN.)
);
#10631=(
NAMED_UNIT(*)
SI_UNIT($,.STERADIAN.)
SOLID_ANGLE_UNIT()
);
#10646=SHAPE_DEFINITION_REPRESENTATION(#10687,#10751);
#10687=PRODUCT_DEFINITION_SHAPE('',$,#10783);
#10751=SHAPE_REPRESENTATION('',(#5519),#10610);
#10768=PRODUCT_DEFINITION_CONTEXT('part definition',#10863,'design');
#10783=PRODUCT_DEFINITION('Cam contact cap','Cam contact cap',#10814,#10768);
#10814=PRODUCT_DEFINITION_FORMATION('',$,#10879);
#10863=APPLICATION_CONTEXT(
'Core Data for Automotive Mechanical Design Process');
#10864=PRODUCT_CONTEXT('part definition',#10863,'mechanical');
#10879=PRODUCT('Cam contact cap','Cam contact cap','Cam contact cap',(#10864));
#10945=COLOUR_RGB('Light Blue',0.38,0.62,0.78);
#10946=FILL_AREA_STYLE_COLOUR('',#10945);
#10947=FILL_AREA_STYLE('',(#10946));
#10948=SURFACE_STYLE_FILL_AREA(#10947);
#10949=SURFACE_SIDE_STYLE('',(#10948));
#10950=SURFACE_STYLE_USAGE(.BOTH.,#10949);
#10951=PRESENTATION_STYLE_ASSIGNMENT((#10950));
ENDSEC;
END-ISO-10303-21;
